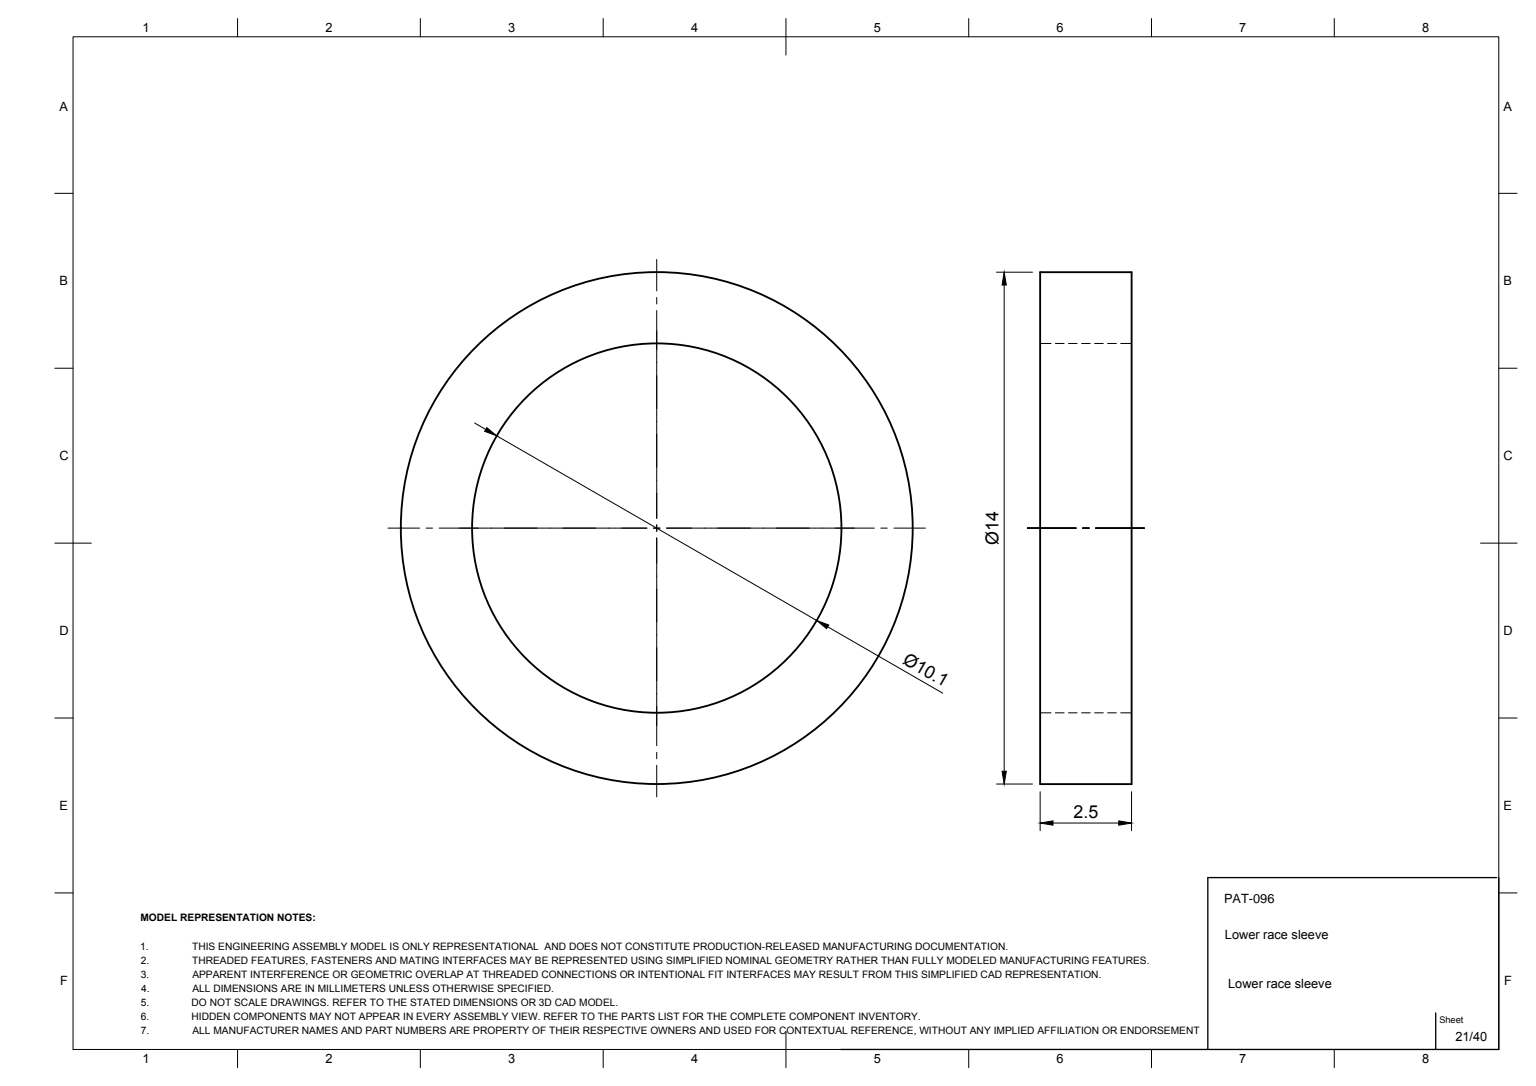
ISO-10303-21;
HEADER;
/* Generated by software containing ST-Developer
 * from STEP Tools, Inc. (www.steptools.com) 
 */

FILE_DESCRIPTION(
/* description */ ('PAT-096'),
/* implementation_level */ '2;1');

FILE_NAME(
/* name */ 'Lower race sleeve.step',
/* time_stamp */ '2026-10-29T17:03:14-07:00',
/* author */ (''),
/* organization */ (''),
/* preprocessor_version */ 'ST-DEVELOPER v20.2',
/* originating_system */ 'Autodesk Translation Framework v15.17.0.0',
/* authorisation */ '');

FILE_SCHEMA (('AUTOMOTIVE_DESIGN { 1 0 10303 214 3 1 1 }'));
ENDSEC;

DATA;
#10=MECHANICAL_DESIGN_GEOMETRIC_PRESENTATION_REPRESENTATION('',(#420),#10650);
#350=SHAPE_REPRESENTATION_RELATIONSHIP('SRR','None',#10812,#381);
#381=ADVANCED_BREP_SHAPE_REPRESENTATION('',(#458),#10630);
#420=STYLED_ITEM('',(#11050),#458);
#458=MANIFOLD_SOLID_BREP('Body1',#5554);
#551=FACE_BOUND('',#1393,.T.);
#552=FACE_BOUND('',#1395,.T.);
#699=PLANE('',#6334);
#700=PLANE('',#6335);
#976=FACE_OUTER_BOUND('',#1390,.T.);
#977=FACE_OUTER_BOUND('',#1391,.T.);
#978=FACE_OUTER_BOUND('',#1392,.T.);
#979=FACE_OUTER_BOUND('',#1394,.T.);
#1390=EDGE_LOOP('',(#4505,#4506,#4507,#4508));
#1391=EDGE_LOOP('',(#4509,#4510,#4511,#4512));
#1392=EDGE_LOOP('',(#4513));
#1393=EDGE_LOOP('',(#4514));
#1394=EDGE_LOOP('',(#4515));
#1395=EDGE_LOOP('',(#4516));
#1767=LINE('',#9818,#2096);
#1768=LINE('',#9824,#2097);
#2096=VECTOR('',#7667,0.505);
#2097=VECTOR('',#7674,0.7);
#2462=CIRCLE('',#6329,0.505);
#2463=CIRCLE('',#6330,0.505);
#2464=CIRCLE('',#6332,0.7);
#2465=CIRCLE('',#6333,0.7);
#2849=VERTEX_POINT('',#9815);
#2850=VERTEX_POINT('',#9817);
#2851=VERTEX_POINT('',#9821);
#2852=VERTEX_POINT('',#9823);
#3431=EDGE_CURVE('',#2849,#2849,#2462,.T.);
#3432=EDGE_CURVE('',#2849,#2850,#1767,.T.);
#3433=EDGE_CURVE('',#2850,#2850,#2463,.T.);
#3434=EDGE_CURVE('',#2851,#2851,#2464,.T.);
#3435=EDGE_CURVE('',#2851,#2852,#1768,.T.);
#3436=EDGE_CURVE('',#2852,#2852,#2465,.T.);
#4505=ORIENTED_EDGE('',*,*,#3431,.F.);
#4506=ORIENTED_EDGE('',*,*,#3432,.T.);
#4507=ORIENTED_EDGE('',*,*,#3433,.T.);
#4508=ORIENTED_EDGE('',*,*,#3432,.F.);
#4509=ORIENTED_EDGE('',*,*,#3434,.F.);
#4510=ORIENTED_EDGE('',*,*,#3435,.T.);
#4511=ORIENTED_EDGE('',*,*,#3436,.T.);
#4512=ORIENTED_EDGE('',*,*,#3435,.F.);
#4513=ORIENTED_EDGE('',*,*,#3434,.T.);
#4514=ORIENTED_EDGE('',*,*,#3431,.T.);
#4515=ORIENTED_EDGE('',*,*,#3436,.F.);
#4516=ORIENTED_EDGE('',*,*,#3433,.F.);
#5144=CYLINDRICAL_SURFACE('',#6328,0.505);
#5145=CYLINDRICAL_SURFACE('',#6331,0.7);
#5381=ADVANCED_FACE('',(#976),#5144,.F.);
#5382=ADVANCED_FACE('',(#977),#5145,.T.);
#5383=ADVANCED_FACE('',(#978,#551),#699,.T.);
#5384=ADVANCED_FACE('',(#979,#552),#700,.F.);
#5554=CLOSED_SHELL('',(#5381,#5382,#5383,#5384));
#6327=AXIS2_PLACEMENT_3D('',#9813,#7661,#7662);
#6328=AXIS2_PLACEMENT_3D('',#9814,#7663,#7664);
#6329=AXIS2_PLACEMENT_3D('',#9816,#7665,#7666);
#6330=AXIS2_PLACEMENT_3D('',#9819,#7668,#7669);
#6331=AXIS2_PLACEMENT_3D('',#9820,#7670,#7671);
#6332=AXIS2_PLACEMENT_3D('',#9822,#7672,#7673);
#6333=AXIS2_PLACEMENT_3D('',#9825,#7675,#7676);
#6334=AXIS2_PLACEMENT_3D('',#9826,#7677,#7678);
#6335=AXIS2_PLACEMENT_3D('',#9827,#7679,#7680);
#7661=DIRECTION('axis',(0.,0.,1.));
#7662=DIRECTION('refdir',(1.,0.,0.));
#7663=DIRECTION('center_axis',(0.,0.,1.));
#7664=DIRECTION('ref_axis',(1.,0.,0.));
#7665=DIRECTION('center_axis',(0.,0.,-1.));
#7666=DIRECTION('ref_axis',(1.,0.,0.));
#7667=DIRECTION('',(0.,0.,-1.));
#7668=DIRECTION('center_axis',(0.,0.,-1.));
#7669=DIRECTION('ref_axis',(1.,0.,0.));
#7670=DIRECTION('center_axis',(0.,0.,1.));
#7671=DIRECTION('ref_axis',(1.,0.,0.));
#7672=DIRECTION('center_axis',(0.,0.,1.));
#7673=DIRECTION('ref_axis',(1.,0.,0.));
#7674=DIRECTION('',(0.,0.,-1.));
#7675=DIRECTION('center_axis',(0.,0.,1.));
#7676=DIRECTION('ref_axis',(1.,0.,0.));
#7677=DIRECTION('center_axis',(0.,0.,1.));
#7678=DIRECTION('ref_axis',(1.,0.,0.));
#7679=DIRECTION('center_axis',(0.,0.,1.));
#7680=DIRECTION('ref_axis',(1.,0.,0.));
#9813=CARTESIAN_POINT('',(0.,0.,0.));
#9814=CARTESIAN_POINT('Origin',(0.,0.,1.8));
#9815=CARTESIAN_POINT('',(-0.505,-6.18446633569413E-17,2.05));
#9816=CARTESIAN_POINT('Origin',(0.,0.,2.05));
#9817=CARTESIAN_POINT('',(-0.505,-6.18446633569413E-17,1.8));
#9818=CARTESIAN_POINT('',(-0.505,-6.18446633569413E-17,1.8));
#9819=CARTESIAN_POINT('Origin',(0.,0.,1.8));
#9820=CARTESIAN_POINT('Origin',(0.,0.,1.8));
#9821=CARTESIAN_POINT('',(-0.7,-8.57252759403147E-17,2.05));
#9822=CARTESIAN_POINT('Origin',(0.,0.,2.05));
#9823=CARTESIAN_POINT('',(-0.7,-8.57252759403147E-17,1.8));
#9824=CARTESIAN_POINT('',(-0.7,-8.57252759403147E-17,1.8));
#9825=CARTESIAN_POINT('Origin',(0.,0.,1.8));
#9826=CARTESIAN_POINT('Origin',(0.,0.,2.05));
#9827=CARTESIAN_POINT('Origin',(0.,0.,1.8));
#10591=UNCERTAINTY_MEASURE_WITH_UNIT(LENGTH_MEASURE(0.001),#10651,
'DISTANCE_ACCURACY_VALUE',
'Maximum model space distance between geometric entities at asserted c
onnectivities');
#10611=UNCERTAINTY_MEASURE_WITH_UNIT(LENGTH_MEASURE(0.001),#10651,
'DISTANCE_ACCURACY_VALUE',
'Maximum model space distance between geometric entities at asserted c
onnectivities');
#10630=(
GEOMETRIC_REPRESENTATION_CONTEXT(3)
GLOBAL_UNCERTAINTY_ASSIGNED_CONTEXT((#10591))
GLOBAL_UNIT_ASSIGNED_CONTEXT((#10651,#10653,#10654))
REPRESENTATION_CONTEXT('','3D')
);
#10650=(
GEOMETRIC_REPRESENTATION_CONTEXT(3)
GLOBAL_UNCERTAINTY_ASSIGNED_CONTEXT((#10611))
GLOBAL_UNIT_ASSIGNED_CONTEXT((#10651,#10653,#10654))
REPRESENTATION_CONTEXT('','3D')
);
#10651=(
LENGTH_UNIT()
NAMED_UNIT(*)
SI_UNIT(.CENTI.,.METRE.)
);
#10653=(
NAMED_UNIT(*)
PLANE_ANGLE_UNIT()
SI_UNIT($,.RADIAN.)
);
#10654=(
NAMED_UNIT(*)
SI_UNIT($,.STERADIAN.)
SOLID_ANGLE_UNIT()
);
#10673=SHAPE_DEFINITION_REPRESENTATION(#10716,#10812);
#10716=PRODUCT_DEFINITION_SHAPE('',$,#10851);
#10812=SHAPE_REPRESENTATION('',(#6327),#10630);
#10832=PRODUCT_DEFINITION_CONTEXT('part definition',#10948,'design');
#10851=PRODUCT_DEFINITION('Lower race sleeve','Lower race sleeve',#10889,
#10832);
#10889=PRODUCT_DEFINITION_FORMATION('',$,#10968);
#10948=APPLICATION_CONTEXT(
'Core Data for Automotive Mechanical Design Process');
#10949=PRODUCT_CONTEXT('part definition',#10948,'mechanical');
#10968=PRODUCT('Lower race sleeve','Lower race sleeve',
'Lower race sleeve',(#10949));
#11044=COLOUR_RGB('Light Blue',0.38,0.62,0.78);
#11045=FILL_AREA_STYLE_COLOUR('',#11044);
#11046=FILL_AREA_STYLE('',(#11045));
#11047=SURFACE_STYLE_FILL_AREA(#11046);
#11048=SURFACE_SIDE_STYLE('',(#11047));
#11049=SURFACE_STYLE_USAGE(.BOTH.,#11048);
#11050=PRESENTATION_STYLE_ASSIGNMENT((#11049));
ENDSEC;
END-ISO-10303-21;
